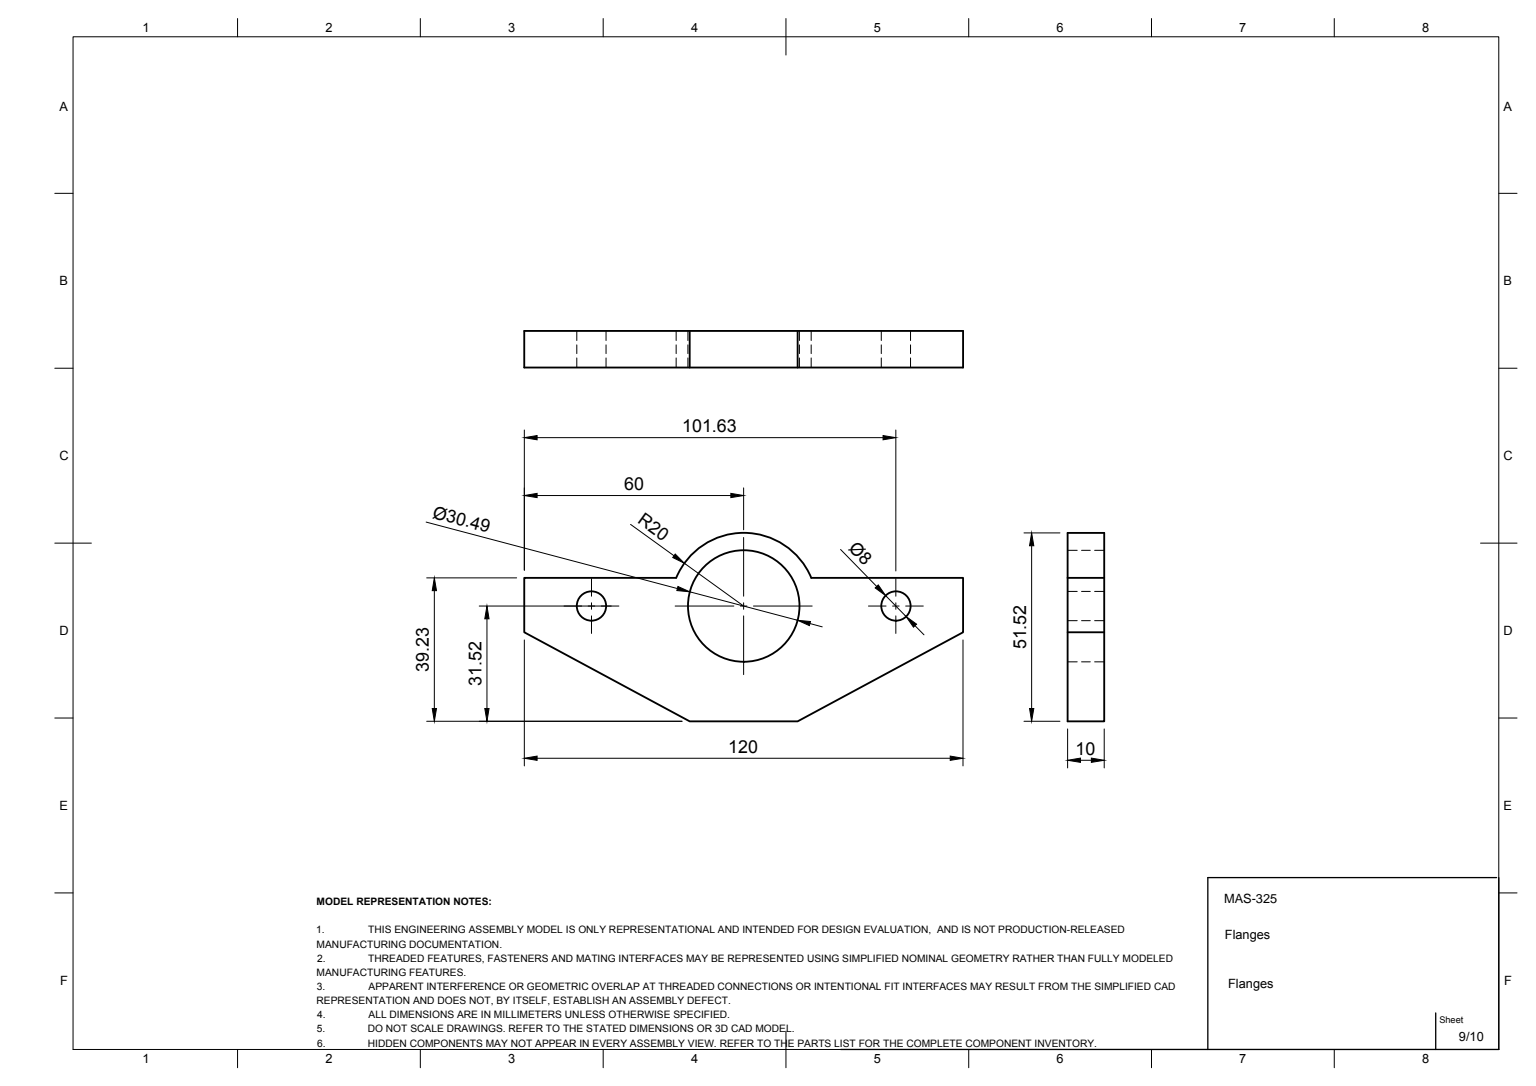
ISO-10303-21;
HEADER;
FILE_DESCRIPTION (('STEP AP214'),
    '1' );
FILE_NAME ('Flanges.step',
    '2026-10-08T01:23:29',
    ( '' ),
    ( '' ),
    'SwSTEP 2.0',
    'SolidWorks 2025',
    '' );
FILE_SCHEMA (( 'AUTOMOTIVE_DESIGN' ));
ENDSEC;

DATA;
#20=AXIS2_PLACEMENT_3D ( 'NONE', #37352, #1353, #33432 ) ;
#23=DIRECTION ( 'NONE',  ( -0.000000000000000000, 1.000000000000000000, -0.000000000000000000 ) ) ;
#63=ORIENTED_EDGE ( 'NONE', *, *, #44474, .F. ) ;
#137=CARTESIAN_POINT ( 'NONE',  ( -180.0000000000000568, -123.5000000000000284, 6.938893903907228378E-15 ) ) ;
#237=CARTESIAN_POINT ( 'NONE',  ( -180.0000000000000568, -115.7896721143442278, 18.45401972188388839 ) ) ;
#349=CARTESIAN_POINT ( 'NONE',  ( -180.0000000000000568, -130.6726371812771959, -60.00000000000000711 ) ) ;
#639=ORIENTED_EDGE ( 'NONE', *, *, #7258, .T. ) ;
#818=CARTESIAN_POINT ( 'NONE',  ( -170.0000000000000284, -123.5000000000000284, -15.24495751795538290 ) ) ;
#819=CARTESIAN_POINT ( 'NONE',  ( -180.0000000000000568, -130.6726371812771959, 60.00000000000000711 ) ) ;
#891=DIRECTION ( 'NONE',  ( -1.000000000000000000, 0.000000000000000000, 0.000000000000000000 ) ) ;
#922=CIRCLE ( 'NONE', #7638, 4.000000000000003553 ) ;
#1076=EDGE_LOOP ( 'NONE', ( #42228, #13718, #8425, #36051 ) ) ;
#1167=CARTESIAN_POINT ( 'NONE',  ( -170.0000000000000284, -115.7896721143442278, 18.45401972188388839 ) ) ;
#1184=ORIENTED_EDGE ( 'NONE', *, *, #26596, .T. ) ;
#1211=VECTOR ( 'NONE', #1937, 1000.000000000000000 ) ;
#1353=DIRECTION ( 'NONE',  ( -1.000000000000000000, 0.000000000000000000, 0.000000000000000000 ) ) ;
#1399=AXIS2_PLACEMENT_3D ( 'NONE', #20888, #36905, #891 ) ;
#1519=FILL_AREA_STYLE_COLOUR ( '', #35988 ) ;
#1546=PLANE ( 'NONE',  #35528 ) ;
#1937=DIRECTION ( 'NONE',  ( -0.000000000000000000, -0.000000000000000000, 1.000000000000000000 ) ) ;
#2726=FACE_OUTER_BOUND ( 'NONE', #33811, .T. ) ;
#3099=VECTOR ( 'NONE', #34479, 1000.000000000000000 ) ;
#3316=DIRECTION ( 'NONE',  ( 1.000000000000000000, -0.000000000000000000, -0.000000000000000000 ) ) ;
#3463=ORIENTED_EDGE ( 'NONE', *, *, #6080, .F. ) ;
#3606=LINE ( 'NONE', #31731, #14611 ) ;
#3613=CARTESIAN_POINT ( 'NONE',  ( -170.0000000000000284, -123.5000000000000284, -37.63467731922663972 ) ) ;
#3664=SHAPE_REPRESENTATION_RELATIONSHIP ( 'NONE' , 'NONE' ,  #24080, #28043 ) ;
#3683=EDGE_CURVE ( 'NONE', #26682, #51653, #46805, .T. ) ;
#3714=CARTESIAN_POINT ( 'NONE',  ( 0.000000000000000000, 0.000000000000000000, 0.000000000000000000 ) ) ;
#3720=AXIS2_PLACEMENT_3D ( 'NONE', #6838, #22864, #30737 ) ;
#3744=ADVANCED_FACE ( 'NONE', ( #30166, #50409, #25703, #5994 ), #5230, .F. ) ;
#4100=CYLINDRICAL_SURFACE ( 'NONE', #13167, 15.24495751795539000 ) ;
#4228=CARTESIAN_POINT ( 'NONE',  ( -170.0000000000000284, -123.5000000000000284, 41.63467731922665394 ) ) ;
#4331=AXIS2_PLACEMENT_3D ( 'NONE', #40308, #20097, #7750 ) ;
#4401=VECTOR ( 'NONE', #12046, 1000.000000000000114 ) ;
#4711=SHAPE_DEFINITION_REPRESENTATION ( #21821, #24080 ) ;
#4811=ORIENTED_EDGE ( 'NONE', *, *, #26596, .F. ) ;
#4908=ORIENTED_EDGE ( 'NONE', *, *, #14096, .F. ) ;
#4947=LINE ( 'NONE', #19100, #13306 ) ;
#5016=ADVANCED_FACE ( 'NONE', ( #35655 ), #42779, .F. ) ;
#5171=( LENGTH_UNIT ( ) NAMED_UNIT ( * ) SI_UNIT ( .MILLI., .METRE. ) );
#5230=PLANE ( 'NONE',  #9884 ) ;
#5370=ADVANCED_FACE ( 'NONE', ( #40305 ), #36373, .F. ) ;
#5401=ORIENTED_EDGE ( 'NONE', *, *, #12187, .F. ) ;
#5503=FACE_OUTER_BOUND ( 'NONE', #30435, .T. ) ;
#5525=CARTESIAN_POINT ( 'NONE',  ( -180.0000000000000568, -123.5000000000000284, -37.63467731922663972 ) ) ;
#5567=CARTESIAN_POINT ( 'NONE',  ( -170.0000000000000284, -123.5000000000000284, 37.63467731922665394 ) ) ;
#5790=VECTOR ( 'NONE', #20175, 1000.000000000000000 ) ;
#5803=EDGE_CURVE ( 'NONE', #7481, #26682, #17665, .T. ) ;
#5824=VERTEX_POINT ( 'NONE', #21332 ) ;
#5994=FACE_BOUND ( 'NONE', #27705, .T. ) ;
#6080=EDGE_CURVE ( 'NONE', #37774, #49603, #11570, .T. ) ;
#6110=CARTESIAN_POINT ( 'NONE',  ( -170.0000000000000284, -123.5000000000000284, 15.24495751795539711 ) ) ;
#6164=VECTOR ( 'NONE', #12329, 1000.000000000000000 ) ;
#6192=CARTESIAN_POINT ( 'NONE',  ( -170.0000000000000284, -115.7896721143442278, -18.45401972188387418 ) ) ;
#6283=DIRECTION ( 'NONE',  ( 0.000000000000000000, 0.000000000000000000, -1.000000000000000000 ) ) ;
#6401=ORIENTED_EDGE ( 'NONE', *, *, #31537, .T. ) ;
#6467=AXIS2_PLACEMENT_3D ( 'NONE', #28761, #16446, #32464 ) ;
#6484=EDGE_LOOP ( 'NONE', ( #15899, #7817, #13656, #8024 ) ) ;
#6614=DIRECTION ( 'NONE',  ( -0.000000000000000000, 0.4739294676984008858, 0.8805628084623552398 ) ) ;
#6646=DIRECTION ( 'NONE',  ( -0.000000000000000000, -0.000000000000000000, -1.000000000000000000 ) ) ;
#6838=CARTESIAN_POINT ( 'NONE',  ( -170.0000000000000284, -123.5000000000000284, 6.938893903907228378E-15 ) ) ;
#6882=VERTEX_POINT ( 'NONE', #26878 ) ;
#6913=CARTESIAN_POINT ( 'NONE',  ( -170.0000000000000284, -155.0173647354142759, 14.76740078976490622 ) ) ;
#6973=CARTESIAN_POINT ( 'NONE',  ( -180.0000000000000568, -123.5000000000000284, 6.938893903907228378E-15 ) ) ;
#7170=LINE ( 'NONE', #48154, #28930 ) ;
#7200=ADVANCED_FACE ( 'NONE', ( #50503 ), #47070, .F. ) ;
#7233=DIRECTION ( 'NONE',  ( -1.000000000000000000, 0.000000000000000000, 0.000000000000000000 ) ) ;
#7254=EDGE_LOOP ( 'NONE', ( #49417, #39039, #23901, #23868 ) ) ;
#7258=EDGE_CURVE ( 'NONE', #17693, #22066, #42601, .T. ) ;
#7481=VERTEX_POINT ( 'NONE', #5525 ) ;
#7638=AXIS2_PLACEMENT_3D ( 'NONE', #13905, #9973, #46480 ) ;
#7644=EDGE_CURVE ( 'NONE', #33465, #47404, #19151, .T. ) ;
#7750=DIRECTION ( 'NONE',  ( 0.000000000000000000, -0.000000000000000000, -1.000000000000000000 ) ) ;
#7817=ORIENTED_EDGE ( 'NONE', *, *, #23921, .T. ) ;
#7870=APPLICATION_CONTEXT ( 'automotive_design' ) ;
#8001=DIRECTION ( 'NONE',  ( -1.000000000000000000, 0.000000000000000000, 0.000000000000000000 ) ) ;
#8024=ORIENTED_EDGE ( 'NONE', *, *, #20853, .F. ) ;
#8143=CARTESIAN_POINT ( 'NONE',  ( -180.0000000000000568, -155.0173647354142759, -14.76740078976489201 ) ) ;
#8304=( GEOMETRIC_REPRESENTATION_CONTEXT ( 3 ) GLOBAL_UNCERTAINTY_ASSIGNED_CONTEXT ( ( #27427 ) ) GLOBAL_UNIT_ASSIGNED_CONTEXT ( ( #5171, #25393, #17526 ) ) REPRESENTATION_CONTEXT ( 'NONE', 'WORKASPACE' ) );
#8381=CARTESIAN_POINT ( 'NONE',  ( -170.0000000000000284, -123.5000000000000284, -41.63467731922663972 ) ) ;
#8425=ORIENTED_EDGE ( 'NONE', *, *, #21696, .F. ) ;
#8438=DIRECTION ( 'NONE',  ( 1.000000000000000000, 0.000000000000000000, 0.000000000000000000 ) ) ;
#8654=ORIENTED_EDGE ( 'NONE', *, *, #19872, .T. ) ;
#8681=EDGE_CURVE ( 'NONE', #17017, #13772, #51453, .T. ) ;
#8709=ADVANCED_FACE ( 'NONE', ( #28026 ), #23337, .F. ) ;
#9066=ORIENTED_EDGE ( 'NONE', *, *, #23675, .F. ) ;
#9208=DIRECTION ( 'NONE',  ( -1.000000000000000000, 0.000000000000000000, 0.000000000000000000 ) ) ;
#9462=AXIS2_PLACEMENT_3D ( 'NONE', #47845, #38903, #35738 ) ;
#9464=FACE_OUTER_BOUND ( 'NONE', #6484, .T. ) ;
#9689=DIRECTION ( 'NONE',  ( 1.000000000000000000, 0.000000000000000000, -0.000000000000000000 ) ) ;
#9813=ORIENTED_EDGE ( 'NONE', *, *, #29055, .T. ) ;
#9837=EDGE_CURVE ( 'NONE', #13772, #5824, #18464, .T. ) ;
#9884=AXIS2_PLACEMENT_3D ( 'NONE', #49377, #34106, #33589 ) ;
#9973=DIRECTION ( 'NONE',  ( -1.000000000000000000, 0.000000000000000000, 0.000000000000000000 ) ) ;
#10082=EDGE_CURVE ( 'NONE', #28841, #17017, #24998, .T. ) ;
#10199=DIRECTION ( 'NONE',  ( 0.000000000000000000, 0.000000000000000000, 1.000000000000000000 ) ) ;
#10618=DIRECTION ( 'NONE',  ( 1.000000000000000000, -0.000000000000000000, -0.000000000000000000 ) ) ;
#10634=CARTESIAN_POINT ( 'NONE',  ( -180.0000000000000568, -123.5000000000000284, 37.63467731922665394 ) ) ;
#10649=VERTEX_POINT ( 'NONE', #16590 ) ;
#10806=ORIENTED_EDGE ( 'NONE', *, *, #26030, .F. ) ;
#10834=CARTESIAN_POINT ( 'NONE',  ( -170.0000000000000284, -115.7896721143442278, -60.00000000000000711 ) ) ;
#10990=DIRECTION ( 'NONE',  ( 1.000000000000000000, -0.000000000000000000, -0.000000000000000000 ) ) ;
#11266=ORIENTED_EDGE ( 'NONE', *, *, #14751, .T. ) ;
#11354=DIRECTION ( 'NONE',  ( 0.000000000000000000, -1.000000000000000000, 0.000000000000000000 ) ) ;
#11432=AXIS2_PLACEMENT_3D ( 'NONE', #17264, #32763, #24612 ) ;
#11453=CYLINDRICAL_SURFACE ( 'NONE', #18818, 4.000000000000003553 ) ;
#11570=LINE ( 'NONE', #8143, #19074 ) ;
#11691=PLANE ( 'NONE',  #4331 ) ;
#11712=EDGE_LOOP ( 'NONE', ( #40945, #3463, #35648, #26863 ) ) ;
#11738=LINE ( 'NONE', #44058, #41347 ) ;
#11918=CARTESIAN_POINT ( 'NONE',  ( -170.0000000000000284, -123.5000000000000284, -45.63467731922664683 ) ) ;
#11932=CARTESIAN_POINT ( 'NONE',  ( -180.0000000000000568, -123.5000000000000284, 41.63467731922665394 ) ) ;
#11970=CARTESIAN_POINT ( 'NONE',  ( -180.0000000000000568, -123.5000000000000284, -41.63467731922663972 ) ) ;
#12046=DIRECTION ( 'NONE',  ( 0.000000000000000000, -0.4739294676984007193, 0.8805628084623552398 ) ) ;
#12187=EDGE_CURVE ( 'NONE', #25065, #34424, #31380, .T. ) ;
#12289=AXIS2_PLACEMENT_3D ( 'NONE', #15482, #27289, #43329 ) ;
#12329=DIRECTION ( 'NONE',  ( -0.000000000000000000, -0.000000000000000000, -1.000000000000000000 ) ) ;
#12377=LINE ( 'NONE', #15831, #30358 ) ;
#12420=VERTEX_POINT ( 'NONE', #37613 ) ;
#12561=EDGE_CURVE ( 'NONE', #25331, #17110, #14477, .T. ) ;
#12690=LINE ( 'NONE', #349, #43254 ) ;
#12842=DIRECTION ( 'NONE',  ( -1.000000000000000000, 0.000000000000000000, 0.000000000000000000 ) ) ;
#13148=DIRECTION ( 'NONE',  ( 0.000000000000000000, 0.000000000000000000, -1.000000000000000000 ) ) ;
#13167=AXIS2_PLACEMENT_3D ( 'NONE', #137, #3316, #36141 ) ;
#13182=ORIENTED_EDGE ( 'NONE', *, *, #8681, .T. ) ;
#13306=VECTOR ( 'NONE', #30386, 1000.000000000000000 ) ;
#13332=STYLED_ITEM ( 'NONE', ( #33004 ), #36851 ) ;
#13378=CARTESIAN_POINT ( 'NONE',  ( -180.0000000000000568, -155.0173647354142759, 14.76740078976490622 ) ) ;
#13464=CARTESIAN_POINT ( 'NONE',  ( -180.0000000000000568, -115.7896721143442278, -18.45401972188387418 ) ) ;
#13544=VERTEX_POINT ( 'NONE', #38665 ) ;
#13656=ORIENTED_EDGE ( 'NONE', *, *, #17988, .F. ) ;
#13661=CARTESIAN_POINT ( 'NONE',  ( -180.0000000000000568, -123.5000000000000284, 41.63467731922665394 ) ) ;
#13718=ORIENTED_EDGE ( 'NONE', *, *, #23233, .F. ) ;
#13724=EDGE_CURVE ( 'NONE', #22066, #47404, #31040, .T. ) ;
#13764=CARTESIAN_POINT ( 'NONE',  ( -180.0000000000000568, -130.6726371812771959, -60.00000000000000711 ) ) ;
#13772=VERTEX_POINT ( 'NONE', #40728 ) ;
#13804=PRODUCT_DEFINITION_CONTEXT ( 'detailed design', #30352, 'design' ) ;
#13823=SURFACE_SIDE_STYLE ('',( #29058 ) ) ;
#13833=EDGE_CURVE ( 'NONE', #12420, #45870, #20585, .T. ) ;
#13905=CARTESIAN_POINT ( 'NONE',  ( -180.0000000000000568, -123.5000000000000284, 41.63467731922665394 ) ) ;
#14096=EDGE_CURVE ( 'NONE', #51653, #26682, #32447, .T. ) ;
#14180=ORIENTED_EDGE ( 'NONE', *, *, #21696, .T. ) ;
#14348=PLANE ( 'NONE',  #48195 ) ;
#14387=VERTEX_POINT ( 'NONE', #10634 ) ;
#14477=LINE ( 'NONE', #41813, #49532 ) ;
#14575=CYLINDRICAL_SURFACE ( 'NONE', #37499, 15.24495751795539000 ) ;
#14611=VECTOR ( 'NONE', #47770, 1000.000000000000000 ) ;
#14619=EDGE_CURVE ( 'NONE', #26773, #34920, #39266, .T. ) ;
#14751=EDGE_CURVE ( 'NONE', #47404, #34424, #46079, .T. ) ;
#14788=CARTESIAN_POINT ( 'NONE',  ( -170.0000000000000284, -115.7896721143442278, 18.45401972188388839 ) ) ;
#14831=VECTOR ( 'NONE', #23185, 1000.000000000000000 ) ;
#14864=DIRECTION ( 'NONE',  ( -1.000000000000000000, 0.000000000000000000, 0.000000000000000000 ) ) ;
#15000=AXIS2_PLACEMENT_3D ( 'NONE', #13661, #32847, #13148 ) ;
#15097=LINE ( 'NONE', #22965, #29166 ) ;
#15302=CARTESIAN_POINT ( 'NONE',  ( -170.0000000000000284, -130.6726371812771959, 60.00000000000000711 ) ) ;
#15317=DIRECTION ( 'NONE',  ( 1.000000000000000000, -0.000000000000000000, -0.000000000000000000 ) ) ;
#15482=CARTESIAN_POINT ( 'NONE',  ( -170.0000000000000284, -123.5000000000000284, -41.63467731922663972 ) ) ;
#15499=LINE ( 'NONE', #51500, #4401 ) ;
#15528=ORIENTED_EDGE ( 'NONE', *, *, #14751, .F. ) ;
#15563=ADVANCED_FACE ( 'NONE', ( #46443 ), #18333, .F. ) ;
#15689=ADVANCED_FACE ( 'NONE', ( #51428 ), #11453, .F. ) ;
#15713=CARTESIAN_POINT ( 'NONE',  ( -180.0000000000000568, -155.0173647354142759, 14.76740078976490622 ) ) ;
#15766=EDGE_CURVE ( 'NONE', #5824, #49603, #28516, .T. ) ;
#15831=CARTESIAN_POINT ( 'NONE',  ( -180.0000000000000568, -130.6726371812771959, 60.00000000000000711 ) ) ;
#15889=DIRECTION ( 'NONE',  ( 1.000000000000000000, -0.000000000000000000, -0.000000000000000000 ) ) ;
#15899=ORIENTED_EDGE ( 'NONE', *, *, #25451, .T. ) ;
#15925=ORIENTED_EDGE ( 'NONE', *, *, #46546, .F. ) ;
#16446=DIRECTION ( 'NONE',  ( -1.000000000000000000, 0.000000000000000000, 0.000000000000000000 ) ) ;
#16589=DIRECTION ( 'NONE',  ( 0.000000000000000000, 0.000000000000000000, 1.000000000000000000 ) ) ;
#16590=CARTESIAN_POINT ( 'NONE',  ( -180.0000000000000568, -123.5000000000000284, -45.63467731922664683 ) ) ;
#17017=VERTEX_POINT ( 'NONE', #40941 ) ;
#17061=DIRECTION ( 'NONE',  ( 0.000000000000000000, 0.000000000000000000, -1.000000000000000000 ) ) ;
#17110=VERTEX_POINT ( 'NONE', #26341 ) ;
#17122=DIRECTION ( 'NONE',  ( 0.000000000000000000, 0.8805628084623552398, -0.4739294676984008858 ) ) ;
#17131=CARTESIAN_POINT ( 'NONE',  ( -170.0000000000000284, -155.0173647354142759, -14.76740078976489201 ) ) ;
#17166=CIRCLE ( 'NONE', #3720, 20.00000000000001776 ) ;
#17264=CARTESIAN_POINT ( 'NONE',  ( -180.0000000000000568, -123.5000000000000284, 6.938893903907228378E-15 ) ) ;
#17366=VERTEX_POINT ( 'NONE', #818 ) ;
#17435=ORIENTED_EDGE ( 'NONE', *, *, #20180, .F. ) ;
#17526=( NAMED_UNIT ( * ) SI_UNIT ( $, .STERADIAN. ) SOLID_ANGLE_UNIT ( ) );
#17606=VECTOR ( 'NONE', #19056, 1000.000000000000000 ) ;
#17665=LINE ( 'NONE', #29994, #23280 ) ;
#17693=VERTEX_POINT ( 'NONE', #39038 ) ;
#17742=VECTOR ( 'NONE', #11354, 1000.000000000000000 ) ;
#17838=ORIENTED_EDGE ( 'NONE', *, *, #12561, .F. ) ;
#17902=AXIS2_PLACEMENT_3D ( 'NONE', #49966, #37620, #29715 ) ;
#17915=DIRECTION ( 'NONE',  ( 1.000000000000000000, -0.000000000000000000, -0.000000000000000000 ) ) ;
#17948=ADVANCED_FACE ( 'NONE', ( #39312 ), #4100, .F. ) ;
#17988=EDGE_CURVE ( 'NONE', #45870, #12420, #29088, .T. ) ;
#18011=VECTOR ( 'NONE', #33768, 1000.000000000000114 ) ;
#18030=CIRCLE ( 'NONE', #48230, 15.24495751795539000 ) ;
#18203=ADVANCED_FACE ( 'NONE', ( #2726 ), #14575, .F. ) ;
#18298=FACE_BOUND ( 'NONE', #25541, .T. ) ;
#18333=PLANE ( 'NONE',  #23023 ) ;
#18464=LINE ( 'NONE', #10834, #14831 ) ;
#18631=AXIS2_PLACEMENT_3D ( 'NONE', #819, #17122, #28918 ) ;
#18818=AXIS2_PLACEMENT_3D ( 'NONE', #11970, #23551, #36151 ) ;
#18853=DIRECTION ( 'NONE',  ( 0.000000000000000000, 0.8805628084623552398, 0.4739294676984007193 ) ) ;
#18926=( NAMED_UNIT ( * ) PLANE_ANGLE_UNIT ( ) SI_UNIT ( $, .RADIAN. ) );
#19056=DIRECTION ( 'NONE',  ( 1.000000000000000000, -0.000000000000000000, -0.000000000000000000 ) ) ;
#19074=VECTOR ( 'NONE', #48351, 1000.000000000000000 ) ;
#19100=CARTESIAN_POINT ( 'NONE',  ( -180.0000000000000568, -123.5000000000000284, 45.63467731922665394 ) ) ;
#19151=LINE ( 'NONE', #35415, #26243 ) ;
#19473=ORIENTED_EDGE ( 'NONE', *, *, #13833, .T. ) ;
#19500=EDGE_LOOP ( 'NONE', ( #45582, #45456, #48409, #41600 ) ) ;
#19612=CARTESIAN_POINT ( 'NONE',  ( -180.0000000000000568, -115.7896721143442278, 60.00000000000000711 ) ) ;
#19671=ORIENTED_EDGE ( 'NONE', *, *, #20853, .T. ) ;
#19707=CARTESIAN_POINT ( 'NONE',  ( -180.0000000000000568, -123.5000000000000284, 6.938893903907228378E-15 ) ) ;
#19721=CARTESIAN_POINT ( 'NONE',  ( -170.0000000000000284, -115.7896721143442278, 60.00000000000000711 ) ) ;
#19807=EDGE_LOOP ( 'NONE', ( #19990, #28047, #24558, #35336 ) ) ;
#19833=FACE_OUTER_BOUND ( 'NONE', #49404, .T. ) ;
#19872=EDGE_CURVE ( 'NONE', #7481, #10649, #37167, .T. ) ;
#19990=ORIENTED_EDGE ( 'NONE', *, *, #14619, .F. ) ;
#19996=ORIENTED_EDGE ( 'NONE', *, *, #43398, .F. ) ;
#20034=MECHANICAL_DESIGN_GEOMETRIC_PRESENTATION_REPRESENTATION('',(#13332),#8304);
#20097=DIRECTION ( 'NONE',  ( 0.000000000000000000, -1.000000000000000000, 0.000000000000000000 ) ) ;
#20175=DIRECTION ( 'NONE',  ( -0.000000000000000000, 1.000000000000000000, -0.000000000000000000 ) ) ;
#20180=EDGE_CURVE ( 'NONE', #33465, #25065, #24954, .T. ) ;
#20446=EDGE_LOOP ( 'NONE', ( #21611, #6401 ) ) ;
#20467=PRODUCT_CONTEXT ( 'NONE', #7870, 'mechanical' ) ;
#20513=ORIENTED_EDGE ( 'NONE', *, *, #5803, .T. ) ;
#20585=CIRCLE ( 'NONE', #25738, 4.000000000000003553 ) ;
#20703=DIRECTION ( 'NONE',  ( -0.000000000000000000, 0.4739294676984008858, 0.8805628084623552398 ) ) ;
#20853=EDGE_CURVE ( 'NONE', #14387, #45870, #50783, .T. ) ;
#20888=CARTESIAN_POINT ( 'NONE',  ( -180.0000000000000568, -115.7896721143442278, 60.00000000000000711 ) ) ;
#20959=PRODUCT ( 'Flanges', 'Flanges', '', ( #20467 ) ) ;
#21262=LINE ( 'NONE', #13378, #43083 ) ;
#21332=CARTESIAN_POINT ( 'NONE',  ( -170.0000000000000284, -130.6726371812771959, -60.00000000000000711 ) ) ;
#21611=ORIENTED_EDGE ( 'NONE', *, *, #23419, .T. ) ;
#21696=EDGE_CURVE ( 'NONE', #25065, #28841, #30864, .T. ) ;
#21753=EDGE_CURVE ( 'NONE', #13544, #17366, #28208, .T. ) ;
#21800=FACE_OUTER_BOUND ( 'NONE', #33500, .T. ) ;
#21810=CARTESIAN_POINT ( 'NONE',  ( -180.0000000000000568, -115.7896721143442278, 18.45401972188388839 ) ) ;
#21821=PRODUCT_DEFINITION_SHAPE ( 'NONE', 'NONE',  #25740 ) ;
#22066=VERTEX_POINT ( 'NONE', #15302 ) ;
#22313=DIRECTION ( 'NONE',  ( 0.000000000000000000, 0.000000000000000000, 1.000000000000000000 ) ) ;
#22324=AXIS2_PLACEMENT_3D ( 'NONE', #50935, #18853, #43553 ) ;
#22536=CARTESIAN_POINT ( 'NONE',  ( -180.0000000000000568, -115.7896721143442278, -18.45401972188387418 ) ) ;
#22621=ORIENTED_EDGE ( 'NONE', *, *, #42085, .F. ) ;
#22711=DIRECTION ( 'NONE',  ( 0.000000000000000000, 0.000000000000000000, -1.000000000000000000 ) ) ;
#22733=CARTESIAN_POINT ( 'NONE',  ( -180.0000000000000568, -115.7896721143442278, 18.45401972188388839 ) ) ;
#22864=DIRECTION ( 'NONE',  ( -1.000000000000000000, 0.000000000000000000, 0.000000000000000000 ) ) ;
#22884=AXIS2_PLACEMENT_3D ( 'NONE', #15713, #31458, #39346 ) ;
#22965=CARTESIAN_POINT ( 'NONE',  ( -180.0000000000000568, -115.7896721143442278, -18.45401972188387418 ) ) ;
#23023=AXIS2_PLACEMENT_3D ( 'NONE', #22536, #26189, #31175 ) ;
#23091=ORIENTED_EDGE ( 'NONE', *, *, #3683, .T. ) ;
#23185=DIRECTION ( 'NONE',  ( 0.000000000000000000, -1.000000000000000000, 0.000000000000000000 ) ) ;
#23233=EDGE_CURVE ( 'NONE', #28841, #51547, #15097, .T. ) ;
#23280=VECTOR ( 'NONE', #17915, 1000.000000000000000 ) ;
#23337=PLANE ( 'NONE',  #22884 ) ;
#23419=EDGE_CURVE ( 'NONE', #17366, #34920, #41821, .T. ) ;
#23545=CIRCLE ( 'NONE', #20, 4.000000000000003553 ) ;
#23551=DIRECTION ( 'NONE',  ( 1.000000000000000000, -0.000000000000000000, -0.000000000000000000 ) ) ;
#23575=DIRECTION ( 'NONE',  ( 1.000000000000000000, -0.000000000000000000, -0.000000000000000000 ) ) ;
#23675=EDGE_CURVE ( 'NONE', #17110, #33465, #27792, .T. ) ;
#23704=VECTOR ( 'NONE', #23575, 1000.000000000000000 ) ;
#23868=ORIENTED_EDGE ( 'NONE', *, *, #23233, .T. ) ;
#23901=ORIENTED_EDGE ( 'NONE', *, *, #10082, .F. ) ;
#23921=EDGE_CURVE ( 'NONE', #6882, #12420, #4947, .T. ) ;
#23987=CIRCLE ( 'NONE', #30700, 4.000000000000003553 ) ;
#24016=ORIENTED_EDGE ( 'NONE', *, *, #19872, .F. ) ;
#24035=DIRECTION ( 'NONE',  ( 0.000000000000000000, 0.000000000000000000, 1.000000000000000000 ) ) ;
#24080=SHAPE_REPRESENTATION ( 'Flanges', ( #31742 ), #49435 ) ;
#24192=EDGE_LOOP ( 'NONE', ( #42089, #19473 ) ) ;
#24558=ORIENTED_EDGE ( 'NONE', *, *, #21753, .T. ) ;
#24612=DIRECTION ( 'NONE',  ( 0.000000000000000000, 0.000000000000000000, 1.000000000000000000 ) ) ;
#24803=ORIENTED_EDGE ( 'NONE', *, *, #45266, .T. ) ;
#24945=DIRECTION ( 'NONE',  ( 0.000000000000000000, 0.000000000000000000, 1.000000000000000000 ) ) ;
#24953=VECTOR ( 'NONE', #26020, 1000.000000000000000 ) ;
#24954=LINE ( 'NONE', #237, #6164 ) ;
#24998=LINE ( 'NONE', #45743, #24953 ) ;
#25065=VERTEX_POINT ( 'NONE', #21810 ) ;
#25106=CARTESIAN_POINT ( 'NONE',  ( -180.0000000000000568, -155.0173647354142759, -14.76740078976489201 ) ) ;
#25157=CARTESIAN_POINT ( 'NONE',  ( -180.0000000000000568, -123.5000000000000284, 15.24495751795539711 ) ) ;
#25326=ORIENTED_EDGE ( 'NONE', *, *, #23675, .T. ) ;
#25331=VERTEX_POINT ( 'NONE', #26153 ) ;
#25393=( NAMED_UNIT ( * ) PLANE_ANGLE_UNIT ( ) SI_UNIT ( $, .RADIAN. ) );
#25451=EDGE_CURVE ( 'NONE', #14387, #6882, #23987, .T. ) ;
#25541=EDGE_LOOP ( 'NONE', ( #10806, #24016 ) ) ;
#25565=ORIENTED_EDGE ( 'NONE', *, *, #7644, .F. ) ;
#25703=FACE_BOUND ( 'NONE', #24192, .T. ) ;
#25738=AXIS2_PLACEMENT_3D ( 'NONE', #4228, #48373, #16589 ) ;
#25740=PRODUCT_DEFINITION ( 'UNKNOWN', '', #44360, #13804 ) ;
#25775=PLANE ( 'NONE',  #18631 ) ;
#26020=DIRECTION ( 'NONE',  ( 0.000000000000000000, 0.000000000000000000, -1.000000000000000000 ) ) ;
#26030=EDGE_CURVE ( 'NONE', #10649, #7481, #23545, .T. ) ;
#26153=CARTESIAN_POINT ( 'NONE',  ( -180.0000000000000568, -155.0173647354142759, 14.76740078976490622 ) ) ;
#26189=DIRECTION ( 'NONE',  ( 0.000000000000000000, -1.000000000000000000, -0.000000000000000000 ) ) ;
#26233=ORIENTED_EDGE ( 'NONE', *, *, #15766, .F. ) ;
#26243=VECTOR ( 'NONE', #10990, 1000.000000000000000 ) ;
#26264=CARTESIAN_POINT ( 'NONE',  ( -170.0000000000000284, -115.7896721143442278, 60.00000000000000711 ) ) ;
#26341=CARTESIAN_POINT ( 'NONE',  ( -180.0000000000000568, -130.6726371812771959, 60.00000000000000711 ) ) ;
#26350=ORIENTED_EDGE ( 'NONE', *, *, #13724, .T. ) ;
#26596=EDGE_CURVE ( 'NONE', #6882, #14387, #922, .T. ) ;
#26682=VERTEX_POINT ( 'NONE', #3613 ) ;
#26773=VERTEX_POINT ( 'NONE', #25157 ) ;
#26863=ORIENTED_EDGE ( 'NONE', *, *, #47879, .T. ) ;
#26878=CARTESIAN_POINT ( 'NONE',  ( -180.0000000000000568, -123.5000000000000284, 45.63467731922665394 ) ) ;
#27058=AXIS2_PLACEMENT_3D ( 'NONE', #19707, #35740, #36012 ) ;
#27072=CIRCLE ( 'NONE', #9462, 15.24495751795539000 ) ;
#27289=DIRECTION ( 'NONE',  ( -1.000000000000000000, 0.000000000000000000, 0.000000000000000000 ) ) ;
#27427=UNCERTAINTY_MEASURE_WITH_UNIT (LENGTH_MEASURE( 1.000000000000000082E-05 ), #5171, 'distance_accuracy_value', 'NONE');
#27439=ORIENTED_EDGE ( 'NONE', *, *, #12561, .T. ) ;
#27705=EDGE_LOOP ( 'NONE', ( #36078, #23091 ) ) ;
#27724=ADVANCED_FACE ( 'NONE', ( #21800 ), #46488, .F. ) ;
#27792=LINE ( 'NONE', #43827, #5790 ) ;
#28026=FACE_OUTER_BOUND ( 'NONE', #19500, .T. ) ;
#28033=ADVANCED_FACE ( 'NONE', ( #47069 ), #43112, .T. ) ;
#28043=ADVANCED_BREP_SHAPE_REPRESENTATION ( '', ( #36851, #31742 ), #49435 ) ;
#28047=ORIENTED_EDGE ( 'NONE', *, *, #50360, .T. ) ;
#28197=DIRECTION ( 'NONE',  ( 1.000000000000000000, -0.000000000000000000, -0.000000000000000000 ) ) ;
#28208=LINE ( 'NONE', #48202, #40822 ) ;
#28220=AXIS2_PLACEMENT_3D ( 'NONE', #34797, #14864, #47419 ) ;
#28331=ORIENTED_EDGE ( 'NONE', *, *, #44833, .T. ) ;
#28341=DIRECTION ( 'NONE',  ( -1.000000000000000000, 0.000000000000000000, 0.000000000000000000 ) ) ;
#28404=DIRECTION ( 'NONE',  ( 1.000000000000000000, -0.000000000000000000, -0.000000000000000000 ) ) ;
#28516=LINE ( 'NONE', #49812, #18011 ) ;
#28761=CARTESIAN_POINT ( 'NONE',  ( -170.0000000000000284, -123.5000000000000284, 41.63467731922665394 ) ) ;
#28793=SURFACE_STYLE_USAGE ( .BOTH. , #13823 ) ;
#28841=VERTEX_POINT ( 'NONE', #13464 ) ;
#28918=DIRECTION ( 'NONE',  ( 0.000000000000000000, 0.4739294676984008858, 0.8805628084623552398 ) ) ;
#28930=VECTOR ( 'NONE', #15317, 1000.000000000000000 ) ;
#29054=ORIENTED_EDGE ( 'NONE', *, *, #20180, .T. ) ;
#29055=EDGE_CURVE ( 'NONE', #25331, #17693, #21262, .T. ) ;
#29058=SURFACE_STYLE_FILL_AREA ( #33576 ) ;
#29087=ADVANCED_FACE ( 'NONE', ( #5503 ), #1546, .F. ) ;
#29088=CIRCLE ( 'NONE', #6467, 4.000000000000003553 ) ;
#29166=VECTOR ( 'NONE', #10618, 1000.000000000000000 ) ;
#29188=ORIENTED_EDGE ( 'NONE', *, *, #26030, .T. ) ;
#29512=ADVANCED_FACE ( 'NONE', ( #50101, #42965, #47184, #18298 ), #14348, .T. ) ;
#29715=DIRECTION ( 'NONE',  ( 0.000000000000000000, 0.000000000000000000, -1.000000000000000000 ) ) ;
#29754=ORIENTED_EDGE ( 'NONE', *, *, #13833, .F. ) ;
#29862=EDGE_CURVE ( 'NONE', #49603, #17693, #46608, .T. ) ;
#29994=CARTESIAN_POINT ( 'NONE',  ( -180.0000000000000568, -123.5000000000000284, -37.63467731922663972 ) ) ;
#30077=DIRECTION ( 'NONE',  ( 1.000000000000000000, -0.000000000000000000, -0.000000000000000000 ) ) ;
#30150=EDGE_CURVE ( 'NONE', #10649, #51653, #7170, .T. ) ;
#30166=FACE_OUTER_BOUND ( 'NONE', #43696, .T. ) ;
#30352=APPLICATION_CONTEXT ( 'automotive_design' ) ;
#30358=VECTOR ( 'NONE', #28404, 1000.000000000000000 ) ;
#30386=DIRECTION ( 'NONE',  ( 1.000000000000000000, -0.000000000000000000, -0.000000000000000000 ) ) ;
#30435=EDGE_LOOP ( 'NONE', ( #37262, #44105, #19996, #13182 ) ) ;
#30579=ORIENTED_EDGE ( 'NONE', *, *, #40435, .F. ) ;
#30700=AXIS2_PLACEMENT_3D ( 'NONE', #11932, #8001, #24035 ) ;
#30737=DIRECTION ( 'NONE',  ( 0.000000000000000000, 0.000000000000000000, 1.000000000000000000 ) ) ;
#30864=CIRCLE ( 'NONE', #28220, 20.00000000000001776 ) ;
#31040=LINE ( 'NONE', #19721, #45395 ) ;
#31175=DIRECTION ( 'NONE',  ( 0.000000000000000000, 0.000000000000000000, -1.000000000000000000 ) ) ;
#31281=DIRECTION ( 'NONE',  ( 1.000000000000000000, -0.000000000000000000, -0.000000000000000000 ) ) ;
#31329=LINE ( 'NONE', #43682, #17742 ) ;
#31380=LINE ( 'NONE', #22733, #17606 ) ;
#31458=DIRECTION ( 'NONE',  ( 0.000000000000000000, 1.000000000000000000, 0.000000000000000000 ) ) ;
#31537=EDGE_CURVE ( 'NONE', #34920, #17366, #18030, .T. ) ;
#31731=CARTESIAN_POINT ( 'NONE',  ( -170.0000000000000284, -115.7896721143442278, -18.45401972188387418 ) ) ;
#31742=AXIS2_PLACEMENT_3D ( 'NONE', #3714, #31843, #8438 ) ;
#31843=DIRECTION ( 'NONE',  ( 0.000000000000000000, 0.000000000000000000, 1.000000000000000000 ) ) ;
#32447=CIRCLE ( 'NONE', #12289, 4.000000000000003553 ) ;
#32464=DIRECTION ( 'NONE',  ( 0.000000000000000000, 0.000000000000000000, 1.000000000000000000 ) ) ;
#32763=DIRECTION ( 'NONE',  ( -1.000000000000000000, 0.000000000000000000, 0.000000000000000000 ) ) ;
#32847=DIRECTION ( 'NONE',  ( 1.000000000000000000, -0.000000000000000000, -0.000000000000000000 ) ) ;
#33004=PRESENTATION_STYLE_ASSIGNMENT (( #28793 ) ) ;
#33351=DIRECTION ( 'NONE',  ( 1.000000000000000000, -0.000000000000000000, -0.000000000000000000 ) ) ;
#33432=DIRECTION ( 'NONE',  ( 0.000000000000000000, 0.000000000000000000, -1.000000000000000000 ) ) ;
#33465=VERTEX_POINT ( 'NONE', #19612 ) ;
#33500=EDGE_LOOP ( 'NONE', ( #49953, #8654, #35184, #44770 ) ) ;
#33576=FILL_AREA_STYLE ('',( #1519 ) ) ;
#33589=DIRECTION ( 'NONE',  ( 0.000000000000000000, 0.000000000000000000, 1.000000000000000000 ) ) ;
#33768=DIRECTION ( 'NONE',  ( 0.000000000000000000, -0.4739294676984007193, 0.8805628084623552398 ) ) ;
#33811=EDGE_LOOP ( 'NONE', ( #39732, #41917, #40207, #40098 ) ) ;
#34106=DIRECTION ( 'NONE',  ( -1.000000000000000000, 0.000000000000000000, 0.000000000000000000 ) ) ;
#34157=ORIENTED_EDGE ( 'NONE', *, *, #7258, .F. ) ;
#34424=VERTEX_POINT ( 'NONE', #1167 ) ;
#34479=DIRECTION ( 'NONE',  ( 1.000000000000000000, -0.000000000000000000, -0.000000000000000000 ) ) ;
#34797=CARTESIAN_POINT ( 'NONE',  ( -180.0000000000000568, -123.5000000000000284, 6.938893903907228378E-15 ) ) ;
#34920=VERTEX_POINT ( 'NONE', #6110 ) ;
#34941=( NAMED_UNIT ( * ) SI_UNIT ( $, .STERADIAN. ) SOLID_ANGLE_UNIT ( ) );
#35184=ORIENTED_EDGE ( 'NONE', *, *, #30150, .T. ) ;
#35221=ADVANCED_FACE ( 'NONE', ( #9464 ), #45728, .F. ) ;
#35316=CARTESIAN_POINT ( 'NONE',  ( -180.0000000000000568, -123.5000000000000284, 15.24495751795539711 ) ) ;
#35336=ORIENTED_EDGE ( 'NONE', *, *, #31537, .F. ) ;
#35415=CARTESIAN_POINT ( 'NONE',  ( -180.0000000000000568, -115.7896721143442278, 60.00000000000000711 ) ) ;
#35427=VECTOR ( 'NONE', #6614, 1000.000000000000114 ) ;
#35479=CLOSED_SHELL ( 'NONE', ( #15689, #35221, #18203, #29512, #3744, #28033, #15563, #29087, #5016, #8709, #44605, #5370, #44233, #17948, #7200, #27724 ) ) ;
#35528=AXIS2_PLACEMENT_3D ( 'NONE', #45700, #10199, #9689 ) ;
#35648=ORIENTED_EDGE ( 'NONE', *, *, #44833, .F. ) ;
#35655=FACE_OUTER_BOUND ( 'NONE', #11712, .T. ) ;
#35659=CARTESIAN_POINT ( 'NONE',  ( -180.0000000000000568, -115.7896721143442278, -60.00000000000000711 ) ) ;
#35738=DIRECTION ( 'NONE',  ( 0.000000000000000000, 0.000000000000000000, 1.000000000000000000 ) ) ;
#35740=DIRECTION ( 'NONE',  ( 1.000000000000000000, -0.000000000000000000, -0.000000000000000000 ) ) ;
#35988=COLOUR_RGB ( '', 0.40784314, 0.44705882, 0.49803922) ;
#36012=DIRECTION ( 'NONE',  ( 0.000000000000000000, 0.000000000000000000, -1.000000000000000000 ) ) ;
#36018=ORIENTED_EDGE ( 'NONE', *, *, #7644, .T. ) ;
#36051=ORIENTED_EDGE ( 'NONE', *, *, #12187, .T. ) ;
#36078=ORIENTED_EDGE ( 'NONE', *, *, #14096, .T. ) ;
#36141=DIRECTION ( 'NONE',  ( 0.000000000000000000, 0.000000000000000000, -1.000000000000000000 ) ) ;
#36151=DIRECTION ( 'NONE',  ( 0.000000000000000000, 0.000000000000000000, -1.000000000000000000 ) ) ;
#36373=PLANE ( 'NONE',  #1399 ) ;
#36851=MANIFOLD_SOLID_BREP ( 'Boss-Extrude11', #35479 ) ;
#36905=DIRECTION ( 'NONE',  ( -0.000000000000000000, 0.000000000000000000, -1.000000000000000000 ) ) ;
#37167=CIRCLE ( 'NONE', #17902, 4.000000000000003553 ) ;
#37262=ORIENTED_EDGE ( 'NONE', *, *, #9837, .T. ) ;
#37332=FACE_OUTER_BOUND ( 'NONE', #41031, .T. ) ;
#37352=CARTESIAN_POINT ( 'NONE',  ( -180.0000000000000568, -123.5000000000000284, -41.63467731922663972 ) ) ;
#37499=AXIS2_PLACEMENT_3D ( 'NONE', #41903, #30077, #22711 ) ;
#37613=CARTESIAN_POINT ( 'NONE',  ( -170.0000000000000284, -123.5000000000000284, 45.63467731922665394 ) ) ;
#37620=DIRECTION ( 'NONE',  ( -1.000000000000000000, 0.000000000000000000, 0.000000000000000000 ) ) ;
#37654=EDGE_LOOP ( 'NONE', ( #45607, #4811 ) ) ;
#37774=VERTEX_POINT ( 'NONE', #25106 ) ;
#38146=EDGE_LOOP ( 'NONE', ( #14180, #48244, #51310, #28331, #24803, #27439, #25326, #29054 ) ) ;
#38246=DIRECTION ( 'NONE',  ( 0.000000000000000000, 0.000000000000000000, 1.000000000000000000 ) ) ;
#38593=DIRECTION ( 'NONE',  ( 1.000000000000000000, -0.000000000000000000, -0.000000000000000000 ) ) ;
#38665=CARTESIAN_POINT ( 'NONE',  ( -180.0000000000000568, -123.5000000000000284, -15.24495751795538290 ) ) ;
#38760=AXIS2_PLACEMENT_3D ( 'NONE', #49913, #38593, #6283 ) ;
#38903=DIRECTION ( 'NONE',  ( -1.000000000000000000, 0.000000000000000000, 0.000000000000000000 ) ) ;
#38930=CARTESIAN_POINT ( 'NONE',  ( -180.0000000000000568, -123.5000000000000284, 37.63467731922665394 ) ) ;
#39038=CARTESIAN_POINT ( 'NONE',  ( -170.0000000000000284, -155.0173647354142759, 14.76740078976490622 ) ) ;
#39039=ORIENTED_EDGE ( 'NONE', *, *, #8681, .F. ) ;
#39266=LINE ( 'NONE', #35316, #44099 ) ;
#39312=FACE_OUTER_BOUND ( 'NONE', #19807, .T. ) ;
#39346=DIRECTION ( 'NONE',  ( 0.000000000000000000, -0.000000000000000000, 1.000000000000000000 ) ) ;
#39423=CARTESIAN_POINT ( 'NONE',  ( -180.0000000000000568, -123.5000000000000284, 41.63467731922665394 ) ) ;
#39732=ORIENTED_EDGE ( 'NONE', *, *, #40435, .T. ) ;
#40098=ORIENTED_EDGE ( 'NONE', *, *, #21753, .F. ) ;
#40207=ORIENTED_EDGE ( 'NONE', *, *, #23419, .F. ) ;
#40305=FACE_OUTER_BOUND ( 'NONE', #45821, .T. ) ;
#40308=CARTESIAN_POINT ( 'NONE',  ( -180.0000000000000568, -115.7896721143442278, 18.45401972188388839 ) ) ;
#40435=EDGE_CURVE ( 'NONE', #13544, #26773, #27072, .T. ) ;
#40720=EDGE_LOOP ( 'NONE', ( #30579, #50818 ) ) ;
#40728=CARTESIAN_POINT ( 'NONE',  ( -170.0000000000000284, -115.7896721143442278, -60.00000000000000711 ) ) ;
#40822=VECTOR ( 'NONE', #48721, 1000.000000000000000 ) ;
#40941=CARTESIAN_POINT ( 'NONE',  ( -180.0000000000000568, -115.7896721143442278, -60.00000000000000711 ) ) ;
#40945=ORIENTED_EDGE ( 'NONE', *, *, #15766, .T. ) ;
#40959=CARTESIAN_POINT ( 'NONE',  ( -170.0000000000000284, -123.5000000000000284, 6.938893903907228378E-15 ) ) ;
#41031=EDGE_LOOP ( 'NONE', ( #639, #63, #17838, #9813 ) ) ;
#41347=VECTOR ( 'NONE', #51702, 1000.000000000000000 ) ;
#41600=ORIENTED_EDGE ( 'NONE', *, *, #6080, .T. ) ;
#41616=EDGE_LOOP ( 'NONE', ( #29188, #20513, #4908, #51462 ) ) ;
#41813=CARTESIAN_POINT ( 'NONE',  ( -180.0000000000000568, -130.6726371812771959, 60.00000000000000711 ) ) ;
#41821=CIRCLE ( 'NONE', #48548, 15.24495751795539000 ) ;
#41903=CARTESIAN_POINT ( 'NONE',  ( -180.0000000000000568, -123.5000000000000284, 6.938893903907228378E-15 ) ) ;
#41917=ORIENTED_EDGE ( 'NONE', *, *, #14619, .T. ) ;
#42085=EDGE_CURVE ( 'NONE', #34424, #51547, #17166, .T. ) ;
#42089=ORIENTED_EDGE ( 'NONE', *, *, #17988, .T. ) ;
#42228=ORIENTED_EDGE ( 'NONE', *, *, #42085, .T. ) ;
#42601=LINE ( 'NONE', #50755, #35427 ) ;
#42779=PLANE ( 'NONE',  #22324 ) ;
#42965=FACE_OUTER_BOUND ( 'NONE', #38146, .T. ) ;
#43083=VECTOR ( 'NONE', #33351, 1000.000000000000000 ) ;
#43112=CYLINDRICAL_SURFACE ( 'NONE', #27058, 20.00000000000001776 ) ;
#43115=ORIENTED_EDGE ( 'NONE', *, *, #9837, .F. ) ;
#43254=VECTOR ( 'NONE', #15889, 1000.000000000000000 ) ;
#43316=VERTEX_POINT ( 'NONE', #13764 ) ;
#43329=DIRECTION ( 'NONE',  ( 0.000000000000000000, 0.000000000000000000, -1.000000000000000000 ) ) ;
#43385=DIRECTION ( 'NONE',  ( 0.000000000000000000, 0.000000000000000000, -1.000000000000000000 ) ) ;
#43398=EDGE_CURVE ( 'NONE', #17017, #43316, #31329, .T. ) ;
#43553=DIRECTION ( 'NONE',  ( 0.000000000000000000, -0.4739294676984007193, 0.8805628084623552398 ) ) ;
#43682=CARTESIAN_POINT ( 'NONE',  ( -180.0000000000000568, -115.7896721143442278, -60.00000000000000711 ) ) ;
#43696=EDGE_LOOP ( 'NONE', ( #22621, #15528, #50393, #34157, #48625, #26233, #43115, #15925 ) ) ;
#43827=CARTESIAN_POINT ( 'NONE',  ( -180.0000000000000568, -115.7896721143442278, 60.00000000000000711 ) ) ;
#44058=CARTESIAN_POINT ( 'NONE',  ( -180.0000000000000568, -155.0173647354142759, 14.76740078976490622 ) ) ;
#44099=VECTOR ( 'NONE', #28197, 1000.000000000000000 ) ;
#44105=ORIENTED_EDGE ( 'NONE', *, *, #47879, .F. ) ;
#44130=( LENGTH_UNIT ( ) NAMED_UNIT ( * ) SI_UNIT ( .MILLI., .METRE. ) );
#44233=ADVANCED_FACE ( 'NONE', ( #19833 ), #11691, .F. ) ;
#44360=PRODUCT_DEFINITION_FORMATION_WITH_SPECIFIED_SOURCE ( 'ANY', '', #20959, .NOT_KNOWN. ) ;
#44455=ORIENTED_EDGE ( 'NONE', *, *, #23921, .F. ) ;
#44474=EDGE_CURVE ( 'NONE', #17110, #22066, #12377, .T. ) ;
#44605=ADVANCED_FACE ( 'NONE', ( #37332 ), #25775, .F. ) ;
#44614=ORIENTED_EDGE ( 'NONE', *, *, #44474, .T. ) ;
#44770=ORIENTED_EDGE ( 'NONE', *, *, #3683, .F. ) ;
#44833=EDGE_CURVE ( 'NONE', #43316, #37774, #15499, .T. ) ;
#45266=EDGE_CURVE ( 'NONE', #37774, #25331, #11738, .T. ) ;
#45395=VECTOR ( 'NONE', #23, 1000.000000000000000 ) ;
#45456=ORIENTED_EDGE ( 'NONE', *, *, #29055, .F. ) ;
#45582=ORIENTED_EDGE ( 'NONE', *, *, #29862, .T. ) ;
#45607=ORIENTED_EDGE ( 'NONE', *, *, #25451, .F. ) ;
#45700=CARTESIAN_POINT ( 'NONE',  ( -180.0000000000000568, -115.7896721143442278, -60.00000000000000711 ) ) ;
#45728=CYLINDRICAL_SURFACE ( 'NONE', #15000, 4.000000000000003553 ) ;
#45743=CARTESIAN_POINT ( 'NONE',  ( -180.0000000000000568, -115.7896721143442278, -18.45401972188387418 ) ) ;
#45821=EDGE_LOOP ( 'NONE', ( #26350, #25565, #9066, #44614 ) ) ;
#45870=VERTEX_POINT ( 'NONE', #5567 ) ;
#46079=LINE ( 'NONE', #14788, #47314 ) ;
#46377=AXIS2_PLACEMENT_3D ( 'NONE', #39423, #31281, #43385 ) ;
#46443=FACE_OUTER_BOUND ( 'NONE', #7254, .T. ) ;
#46480=DIRECTION ( 'NONE',  ( 0.000000000000000000, 0.000000000000000000, 1.000000000000000000 ) ) ;
#46488=CYLINDRICAL_SURFACE ( 'NONE', #38760, 4.000000000000003553 ) ;
#46546=EDGE_CURVE ( 'NONE', #51547, #13772, #3606, .T. ) ;
#46608=LINE ( 'NONE', #6913, #1211 ) ;
#46805=CIRCLE ( 'NONE', #51014, 4.000000000000003553 ) ;
#47069=FACE_OUTER_BOUND ( 'NONE', #1076, .T. ) ;
#47070=CYLINDRICAL_SURFACE ( 'NONE', #46377, 4.000000000000003553 ) ;
#47184=FACE_BOUND ( 'NONE', #40720, .T. ) ;
#47314=VECTOR ( 'NONE', #6646, 1000.000000000000000 ) ;
#47404=VERTEX_POINT ( 'NONE', #26264 ) ;
#47419=DIRECTION ( 'NONE',  ( 0.000000000000000000, 0.000000000000000000, 1.000000000000000000 ) ) ;
#47770=DIRECTION ( 'NONE',  ( 0.000000000000000000, 0.000000000000000000, -1.000000000000000000 ) ) ;
#47845=CARTESIAN_POINT ( 'NONE',  ( -180.0000000000000568, -123.5000000000000284, 6.938893903907228378E-15 ) ) ;
#47879=EDGE_CURVE ( 'NONE', #43316, #5824, #12690, .T. ) ;
#48154=CARTESIAN_POINT ( 'NONE',  ( -180.0000000000000568, -123.5000000000000284, -45.63467731922664683 ) ) ;
#48195=AXIS2_PLACEMENT_3D ( 'NONE', #6973, #7233, #38246 ) ;
#48202=CARTESIAN_POINT ( 'NONE',  ( -180.0000000000000568, -123.5000000000000284, -15.24495751795538290 ) ) ;
#48230=AXIS2_PLACEMENT_3D ( 'NONE', #40959, #12842, #24945 ) ;
#48244=ORIENTED_EDGE ( 'NONE', *, *, #10082, .T. ) ;
#48351=DIRECTION ( 'NONE',  ( 1.000000000000000000, -0.000000000000000000, -0.000000000000000000 ) ) ;
#48365=CIRCLE ( 'NONE', #11432, 15.24495751795539000 ) ;
#48373=DIRECTION ( 'NONE',  ( -1.000000000000000000, 0.000000000000000000, 0.000000000000000000 ) ) ;
#48409=ORIENTED_EDGE ( 'NONE', *, *, #45266, .F. ) ;
#48548=AXIS2_PLACEMENT_3D ( 'NONE', #49924, #9208, #22313 ) ;
#48625=ORIENTED_EDGE ( 'NONE', *, *, #29862, .F. ) ;
#48721=DIRECTION ( 'NONE',  ( 1.000000000000000000, -0.000000000000000000, -0.000000000000000000 ) ) ;
#49377=CARTESIAN_POINT ( 'NONE',  ( -170.0000000000000284, -123.5000000000000284, 6.938893903907228378E-15 ) ) ;
#49404=EDGE_LOOP ( 'NONE', ( #11266, #5401, #17435, #36018 ) ) ;
#49417=ORIENTED_EDGE ( 'NONE', *, *, #46546, .T. ) ;
#49435=( GEOMETRIC_REPRESENTATION_CONTEXT ( 3 ) GLOBAL_UNCERTAINTY_ASSIGNED_CONTEXT ( ( #51612 ) ) GLOBAL_UNIT_ASSIGNED_CONTEXT ( ( #44130, #18926, #34941 ) ) REPRESENTATION_CONTEXT ( 'NONE', 'WORKASPACE' ) );
#49532=VECTOR ( 'NONE', #20703, 1000.000000000000114 ) ;
#49603=VERTEX_POINT ( 'NONE', #17131 ) ;
#49812=CARTESIAN_POINT ( 'NONE',  ( -170.0000000000000284, -130.6726371812771959, -60.00000000000000711 ) ) ;
#49913=CARTESIAN_POINT ( 'NONE',  ( -180.0000000000000568, -123.5000000000000284, -41.63467731922663972 ) ) ;
#49924=CARTESIAN_POINT ( 'NONE',  ( -170.0000000000000284, -123.5000000000000284, 6.938893903907228378E-15 ) ) ;
#49953=ORIENTED_EDGE ( 'NONE', *, *, #5803, .F. ) ;
#49966=CARTESIAN_POINT ( 'NONE',  ( -180.0000000000000568, -123.5000000000000284, -41.63467731922663972 ) ) ;
#50101=FACE_BOUND ( 'NONE', #37654, .T. ) ;
#50360=EDGE_CURVE ( 'NONE', #26773, #13544, #48365, .T. ) ;
#50393=ORIENTED_EDGE ( 'NONE', *, *, #13724, .F. ) ;
#50409=FACE_BOUND ( 'NONE', #20446, .T. ) ;
#50503=FACE_OUTER_BOUND ( 'NONE', #51039, .T. ) ;
#50755=CARTESIAN_POINT ( 'NONE',  ( -170.0000000000000284, -130.6726371812771959, 60.00000000000000711 ) ) ;
#50783=LINE ( 'NONE', #38930, #3099 ) ;
#50818=ORIENTED_EDGE ( 'NONE', *, *, #50360, .F. ) ;
#50935=CARTESIAN_POINT ( 'NONE',  ( -180.0000000000000568, -130.6726371812771959, -60.00000000000000711 ) ) ;
#51014=AXIS2_PLACEMENT_3D ( 'NONE', #8381, #28341, #17061 ) ;
#51039=EDGE_LOOP ( 'NONE', ( #44455, #1184, #19671, #29754 ) ) ;
#51310=ORIENTED_EDGE ( 'NONE', *, *, #43398, .T. ) ;
#51428=FACE_OUTER_BOUND ( 'NONE', #41616, .T. ) ;
#51453=LINE ( 'NONE', #35659, #23704 ) ;
#51462=ORIENTED_EDGE ( 'NONE', *, *, #30150, .F. ) ;
#51500=CARTESIAN_POINT ( 'NONE',  ( -180.0000000000000568, -130.6726371812771959, -60.00000000000000711 ) ) ;
#51547=VERTEX_POINT ( 'NONE', #6192 ) ;
#51612=UNCERTAINTY_MEASURE_WITH_UNIT (LENGTH_MEASURE( 1.000000000000000082E-05 ), #44130, 'distance_accuracy_value', 'NONE');
#51653=VERTEX_POINT ( 'NONE', #11918 ) ;
#51702=DIRECTION ( 'NONE',  ( -0.000000000000000000, -0.000000000000000000, 1.000000000000000000 ) ) ;
ENDSEC;
END-ISO-10303-21;
